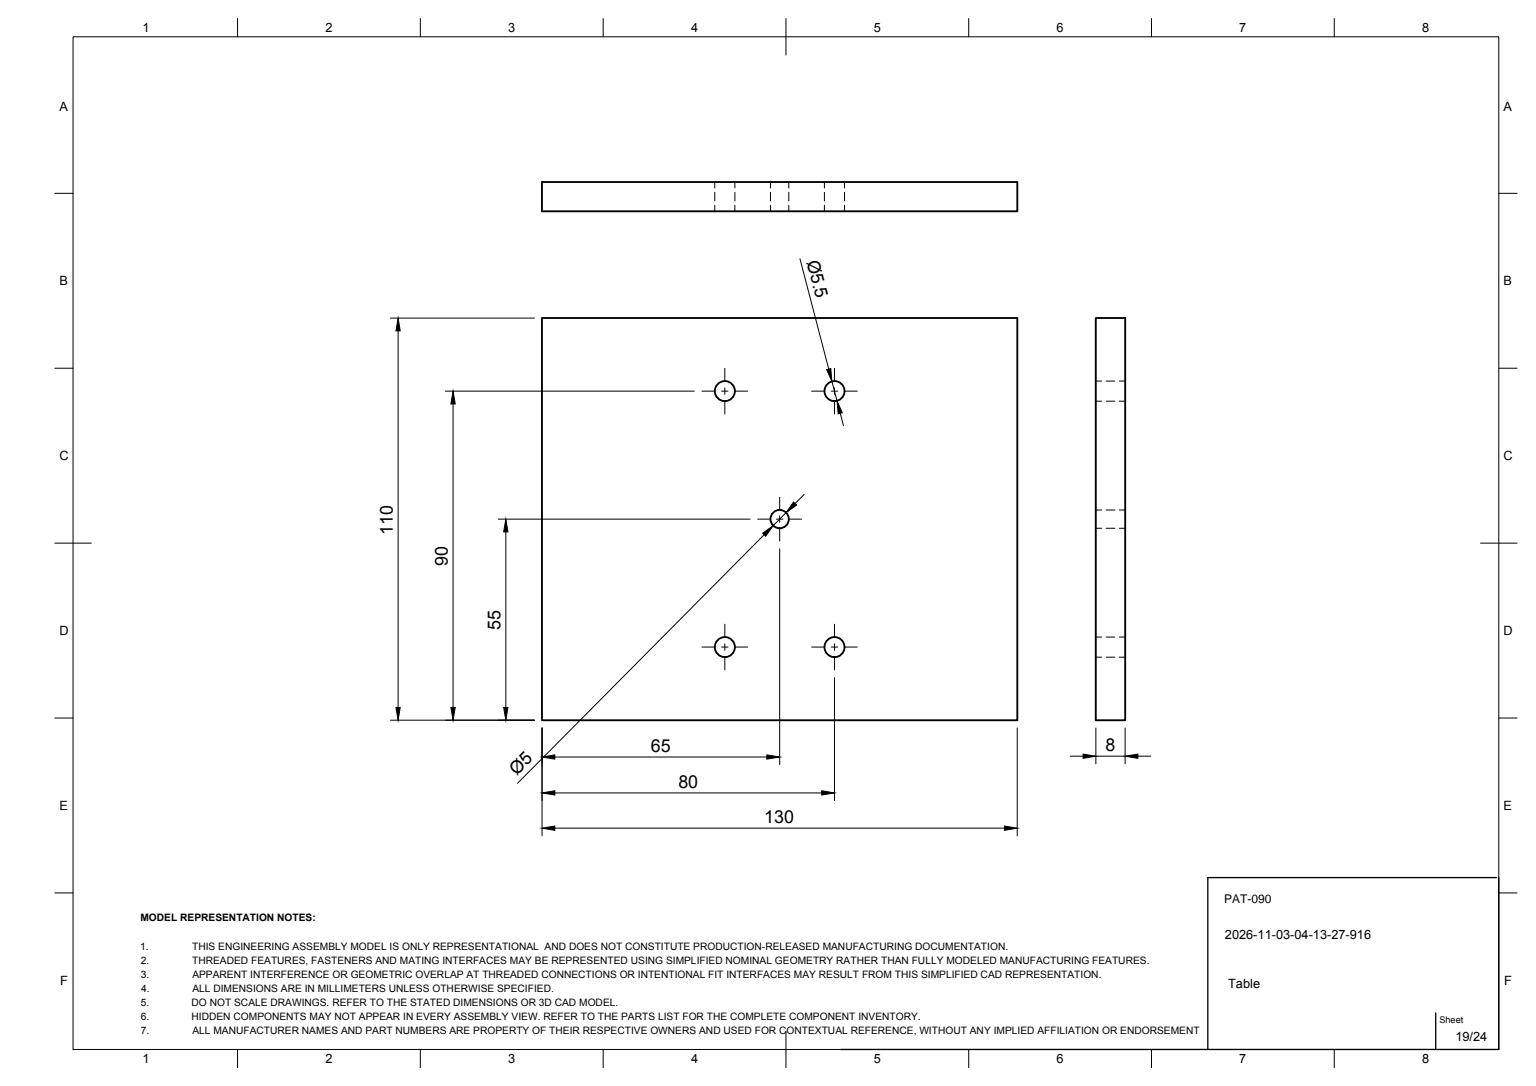
ISO-10303-21;
HEADER;
/* Generated by software containing ST-Developer
 * from STEP Tools, Inc. (www.steptools.com) 
 */

FILE_DESCRIPTION(
/* description */ ('Round-Shaft Linear Stage with Ball Bushings'),
/* implementation_level */ '2;1');

FILE_NAME(
/* name */ 'Table.step',
/* time_stamp */ '2026-10-27T10:47:55-07:00',
/* author */ (''),
/* organization */ (''),
/* preprocessor_version */ 'ST-DEVELOPER v20.2',
/* originating_system */ 'Autodesk Translation Framework v15.17.0.0',
/* authorisation */ '');

FILE_SCHEMA (('AUTOMOTIVE_DESIGN { 1 0 10303 214 3 1 1 }'));
ENDSEC;

DATA;
#10=MECHANICAL_DESIGN_GEOMETRIC_PRESENTATION_REPRESENTATION('',(#315),#7835);
#273=SHAPE_REPRESENTATION_RELATIONSHIP('SRR','None',#7962,#294);
#294=ADVANCED_BREP_SHAPE_REPRESENTATION('',(#335),#7826);
#315=STYLED_ITEM('',(#8158),#335);
#335=MANIFOLD_SOLID_BREP('Body1',#4406);
#431=FACE_BOUND('',#1136,.T.);
#432=FACE_BOUND('',#1137,.T.);
#433=FACE_BOUND('',#1138,.T.);
#434=FACE_BOUND('',#1139,.T.);
#435=FACE_BOUND('',#1140,.T.);
#436=FACE_BOUND('',#1142,.T.);
#437=FACE_BOUND('',#1143,.T.);
#438=FACE_BOUND('',#1144,.T.);
#439=FACE_BOUND('',#1145,.T.);
#440=FACE_BOUND('',#1146,.T.);
#556=PLANE('',#4968);
#557=PLANE('',#4969);
#558=PLANE('',#4970);
#559=PLANE('',#4971);
#560=PLANE('',#4972);
#561=PLANE('',#4973);
#778=FACE_OUTER_BOUND('',#1126,.T.);
#779=FACE_OUTER_BOUND('',#1127,.T.);
#780=FACE_OUTER_BOUND('',#1128,.T.);
#781=FACE_OUTER_BOUND('',#1129,.T.);
#782=FACE_OUTER_BOUND('',#1130,.T.);
#783=FACE_OUTER_BOUND('',#1131,.T.);
#784=FACE_OUTER_BOUND('',#1132,.T.);
#785=FACE_OUTER_BOUND('',#1133,.T.);
#786=FACE_OUTER_BOUND('',#1134,.T.);
#787=FACE_OUTER_BOUND('',#1135,.T.);
#788=FACE_OUTER_BOUND('',#1141,.T.);
#1126=EDGE_LOOP('',(#3686,#3687,#3688,#3689));
#1127=EDGE_LOOP('',(#3690,#3691,#3692,#3693));
#1128=EDGE_LOOP('',(#3694,#3695,#3696,#3697));
#1129=EDGE_LOOP('',(#3698,#3699,#3700,#3701));
#1130=EDGE_LOOP('',(#3702,#3703,#3704,#3705));
#1131=EDGE_LOOP('',(#3706,#3707,#3708,#3709));
#1132=EDGE_LOOP('',(#3710,#3711,#3712,#3713));
#1133=EDGE_LOOP('',(#3714,#3715,#3716,#3717));
#1134=EDGE_LOOP('',(#3718,#3719,#3720,#3721));
#1135=EDGE_LOOP('',(#3722,#3723,#3724,#3725));
#1136=EDGE_LOOP('',(#3726));
#1137=EDGE_LOOP('',(#3727));
#1138=EDGE_LOOP('',(#3728));
#1139=EDGE_LOOP('',(#3729));
#1140=EDGE_LOOP('',(#3730));
#1141=EDGE_LOOP('',(#3731,#3732,#3733,#3734));
#1142=EDGE_LOOP('',(#3735));
#1143=EDGE_LOOP('',(#3736));
#1144=EDGE_LOOP('',(#3737));
#1145=EDGE_LOOP('',(#3738));
#1146=EDGE_LOOP('',(#3739));
#1470=LINE('',#7328,#1810);
#1471=LINE('',#7334,#1811);
#1472=LINE('',#7340,#1812);
#1473=LINE('',#7346,#1813);
#1474=LINE('',#7352,#1814);
#1475=LINE('',#7357,#1815);
#1476=LINE('',#7359,#1816);
#1477=LINE('',#7361,#1817);
#1478=LINE('',#7362,#1818);
#1479=LINE('',#7365,#1819);
#1480=LINE('',#7367,#1820);
#1481=LINE('',#7368,#1821);
#1482=LINE('',#7371,#1822);
#1483=LINE('',#7373,#1823);
#1484=LINE('',#7374,#1824);
#1485=LINE('',#7376,#1825);
#1486=LINE('',#7377,#1826);
#1810=VECTOR('',#6009,0.25);
#1811=VECTOR('',#6016,0.274999999999999);
#1812=VECTOR('',#6023,0.275);
#1813=VECTOR('',#6030,0.275);
#1814=VECTOR('',#6037,0.274999999999999);
#1815=VECTOR('',#6042,1.);
#1816=VECTOR('',#6043,1.);
#1817=VECTOR('',#6044,1.);
#1818=VECTOR('',#6045,1.);
#1819=VECTOR('',#6048,1.);
#1820=VECTOR('',#6049,1.);
#1821=VECTOR('',#6050,1.);
#1822=VECTOR('',#6053,1.);
#1823=VECTOR('',#6054,1.);
#1824=VECTOR('',#6055,1.);
#1825=VECTOR('',#6058,1.);
#1826=VECTOR('',#6059,1.);
#2054=CIRCLE('',#4954,0.25);
#2055=CIRCLE('',#4955,0.25);
#2056=CIRCLE('',#4957,0.274999999999999);
#2057=CIRCLE('',#4958,0.274999999999999);
#2058=CIRCLE('',#4960,0.275);
#2059=CIRCLE('',#4961,0.275);
#2060=CIRCLE('',#4963,0.275);
#2061=CIRCLE('',#4964,0.275);
#2062=CIRCLE('',#4966,0.274999999999999);
#2063=CIRCLE('',#4967,0.274999999999999);
#2347=VERTEX_POINT('',#7325);
#2348=VERTEX_POINT('',#7327);
#2349=VERTEX_POINT('',#7331);
#2350=VERTEX_POINT('',#7333);
#2351=VERTEX_POINT('',#7337);
#2352=VERTEX_POINT('',#7339);
#2353=VERTEX_POINT('',#7343);
#2354=VERTEX_POINT('',#7345);
#2355=VERTEX_POINT('',#7349);
#2356=VERTEX_POINT('',#7351);
#2357=VERTEX_POINT('',#7355);
#2358=VERTEX_POINT('',#7356);
#2359=VERTEX_POINT('',#7358);
#2360=VERTEX_POINT('',#7360);
#2361=VERTEX_POINT('',#7364);
#2362=VERTEX_POINT('',#7366);
#2363=VERTEX_POINT('',#7370);
#2364=VERTEX_POINT('',#7372);
#2811=EDGE_CURVE('',#2347,#2347,#2054,.T.);
#2812=EDGE_CURVE('',#2347,#2348,#1470,.T.);
#2813=EDGE_CURVE('',#2348,#2348,#2055,.T.);
#2814=EDGE_CURVE('',#2349,#2349,#2056,.T.);
#2815=EDGE_CURVE('',#2349,#2350,#1471,.T.);
#2816=EDGE_CURVE('',#2350,#2350,#2057,.T.);
#2817=EDGE_CURVE('',#2351,#2351,#2058,.T.);
#2818=EDGE_CURVE('',#2351,#2352,#1472,.T.);
#2819=EDGE_CURVE('',#2352,#2352,#2059,.T.);
#2820=EDGE_CURVE('',#2353,#2353,#2060,.T.);
#2821=EDGE_CURVE('',#2353,#2354,#1473,.T.);
#2822=EDGE_CURVE('',#2354,#2354,#2061,.T.);
#2823=EDGE_CURVE('',#2355,#2355,#2062,.T.);
#2824=EDGE_CURVE('',#2355,#2356,#1474,.T.);
#2825=EDGE_CURVE('',#2356,#2356,#2063,.T.);
#2826=EDGE_CURVE('',#2357,#2358,#1475,.T.);
#2827=EDGE_CURVE('',#2358,#2359,#1476,.T.);
#2828=EDGE_CURVE('',#2360,#2359,#1477,.T.);
#2829=EDGE_CURVE('',#2357,#2360,#1478,.T.);
#2830=EDGE_CURVE('',#2361,#2357,#1479,.T.);
#2831=EDGE_CURVE('',#2362,#2360,#1480,.T.);
#2832=EDGE_CURVE('',#2361,#2362,#1481,.T.);
#2833=EDGE_CURVE('',#2363,#2361,#1482,.T.);
#2834=EDGE_CURVE('',#2364,#2362,#1483,.T.);
#2835=EDGE_CURVE('',#2363,#2364,#1484,.T.);
#2836=EDGE_CURVE('',#2358,#2363,#1485,.T.);
#2837=EDGE_CURVE('',#2359,#2364,#1486,.T.);
#3686=ORIENTED_EDGE('',*,*,#2811,.F.);
#3687=ORIENTED_EDGE('',*,*,#2812,.T.);
#3688=ORIENTED_EDGE('',*,*,#2813,.F.);
#3689=ORIENTED_EDGE('',*,*,#2812,.F.);
#3690=ORIENTED_EDGE('',*,*,#2814,.F.);
#3691=ORIENTED_EDGE('',*,*,#2815,.T.);
#3692=ORIENTED_EDGE('',*,*,#2816,.F.);
#3693=ORIENTED_EDGE('',*,*,#2815,.F.);
#3694=ORIENTED_EDGE('',*,*,#2817,.F.);
#3695=ORIENTED_EDGE('',*,*,#2818,.T.);
#3696=ORIENTED_EDGE('',*,*,#2819,.F.);
#3697=ORIENTED_EDGE('',*,*,#2818,.F.);
#3698=ORIENTED_EDGE('',*,*,#2820,.F.);
#3699=ORIENTED_EDGE('',*,*,#2821,.T.);
#3700=ORIENTED_EDGE('',*,*,#2822,.F.);
#3701=ORIENTED_EDGE('',*,*,#2821,.F.);
#3702=ORIENTED_EDGE('',*,*,#2823,.F.);
#3703=ORIENTED_EDGE('',*,*,#2824,.T.);
#3704=ORIENTED_EDGE('',*,*,#2825,.F.);
#3705=ORIENTED_EDGE('',*,*,#2824,.F.);
#3706=ORIENTED_EDGE('',*,*,#2826,.T.);
#3707=ORIENTED_EDGE('',*,*,#2827,.T.);
#3708=ORIENTED_EDGE('',*,*,#2828,.F.);
#3709=ORIENTED_EDGE('',*,*,#2829,.F.);
#3710=ORIENTED_EDGE('',*,*,#2830,.T.);
#3711=ORIENTED_EDGE('',*,*,#2829,.T.);
#3712=ORIENTED_EDGE('',*,*,#2831,.F.);
#3713=ORIENTED_EDGE('',*,*,#2832,.F.);
#3714=ORIENTED_EDGE('',*,*,#2833,.T.);
#3715=ORIENTED_EDGE('',*,*,#2832,.T.);
#3716=ORIENTED_EDGE('',*,*,#2834,.F.);
#3717=ORIENTED_EDGE('',*,*,#2835,.F.);
#3718=ORIENTED_EDGE('',*,*,#2836,.T.);
#3719=ORIENTED_EDGE('',*,*,#2835,.T.);
#3720=ORIENTED_EDGE('',*,*,#2837,.F.);
#3721=ORIENTED_EDGE('',*,*,#2827,.F.);
#3722=ORIENTED_EDGE('',*,*,#2837,.T.);
#3723=ORIENTED_EDGE('',*,*,#2834,.T.);
#3724=ORIENTED_EDGE('',*,*,#2831,.T.);
#3725=ORIENTED_EDGE('',*,*,#2828,.T.);
#3726=ORIENTED_EDGE('',*,*,#2813,.T.);
#3727=ORIENTED_EDGE('',*,*,#2816,.T.);
#3728=ORIENTED_EDGE('',*,*,#2819,.T.);
#3729=ORIENTED_EDGE('',*,*,#2822,.T.);
#3730=ORIENTED_EDGE('',*,*,#2825,.T.);
#3731=ORIENTED_EDGE('',*,*,#2836,.F.);
#3732=ORIENTED_EDGE('',*,*,#2826,.F.);
#3733=ORIENTED_EDGE('',*,*,#2830,.F.);
#3734=ORIENTED_EDGE('',*,*,#2833,.F.);
#3735=ORIENTED_EDGE('',*,*,#2811,.T.);
#3736=ORIENTED_EDGE('',*,*,#2814,.T.);
#3737=ORIENTED_EDGE('',*,*,#2817,.T.);
#3738=ORIENTED_EDGE('',*,*,#2820,.T.);
#3739=ORIENTED_EDGE('',*,*,#2823,.T.);
#4112=CYLINDRICAL_SURFACE('',#4953,0.25);
#4113=CYLINDRICAL_SURFACE('',#4956,0.274999999999999);
#4114=CYLINDRICAL_SURFACE('',#4959,0.275);
#4115=CYLINDRICAL_SURFACE('',#4962,0.275);
#4116=CYLINDRICAL_SURFACE('',#4965,0.274999999999999);
#4297=ADVANCED_FACE('',(#778),#4112,.F.);
#4298=ADVANCED_FACE('',(#779),#4113,.F.);
#4299=ADVANCED_FACE('',(#780),#4114,.F.);
#4300=ADVANCED_FACE('',(#781),#4115,.F.);
#4301=ADVANCED_FACE('',(#782),#4116,.F.);
#4302=ADVANCED_FACE('',(#783),#556,.T.);
#4303=ADVANCED_FACE('',(#784),#557,.T.);
#4304=ADVANCED_FACE('',(#785),#558,.T.);
#4305=ADVANCED_FACE('',(#786),#559,.T.);
#4306=ADVANCED_FACE('',(#787,#431,#432,#433,#434,#435),#560,.T.);
#4307=ADVANCED_FACE('',(#788,#436,#437,#438,#439,#440),#561,.F.);
#4406=CLOSED_SHELL('',(#4297,#4298,#4299,#4300,#4301,#4302,#4303,#4304,
#4305,#4306,#4307));
#4952=AXIS2_PLACEMENT_3D('',#7323,#6003,#6004);
#4953=AXIS2_PLACEMENT_3D('',#7324,#6005,#6006);
#4954=AXIS2_PLACEMENT_3D('',#7326,#6007,#6008);
#4955=AXIS2_PLACEMENT_3D('',#7329,#6010,#6011);
#4956=AXIS2_PLACEMENT_3D('',#7330,#6012,#6013);
#4957=AXIS2_PLACEMENT_3D('',#7332,#6014,#6015);
#4958=AXIS2_PLACEMENT_3D('',#7335,#6017,#6018);
#4959=AXIS2_PLACEMENT_3D('',#7336,#6019,#6020);
#4960=AXIS2_PLACEMENT_3D('',#7338,#6021,#6022);
#4961=AXIS2_PLACEMENT_3D('',#7341,#6024,#6025);
#4962=AXIS2_PLACEMENT_3D('',#7342,#6026,#6027);
#4963=AXIS2_PLACEMENT_3D('',#7344,#6028,#6029);
#4964=AXIS2_PLACEMENT_3D('',#7347,#6031,#6032);
#4965=AXIS2_PLACEMENT_3D('',#7348,#6033,#6034);
#4966=AXIS2_PLACEMENT_3D('',#7350,#6035,#6036);
#4967=AXIS2_PLACEMENT_3D('',#7353,#6038,#6039);
#4968=AXIS2_PLACEMENT_3D('',#7354,#6040,#6041);
#4969=AXIS2_PLACEMENT_3D('',#7363,#6046,#6047);
#4970=AXIS2_PLACEMENT_3D('',#7369,#6051,#6052);
#4971=AXIS2_PLACEMENT_3D('',#7375,#6056,#6057);
#4972=AXIS2_PLACEMENT_3D('',#7378,#6060,#6061);
#4973=AXIS2_PLACEMENT_3D('',#7379,#6062,#6063);
#6003=DIRECTION('axis',(0.,0.,1.));
#6004=DIRECTION('refdir',(1.,0.,0.));
#6005=DIRECTION('center_axis',(0.,0.,1.));
#6006=DIRECTION('ref_axis',(1.,0.,0.));
#6007=DIRECTION('center_axis',(0.,0.,1.));
#6008=DIRECTION('ref_axis',(1.,0.,0.));
#6009=DIRECTION('',(0.,0.,1.));
#6010=DIRECTION('center_axis',(0.,0.,-1.));
#6011=DIRECTION('ref_axis',(1.,0.,0.));
#6012=DIRECTION('center_axis',(0.,0.,1.));
#6013=DIRECTION('ref_axis',(1.,0.,0.));
#6014=DIRECTION('center_axis',(0.,0.,1.));
#6015=DIRECTION('ref_axis',(1.,0.,0.));
#6016=DIRECTION('',(0.,0.,1.));
#6017=DIRECTION('center_axis',(0.,0.,-1.));
#6018=DIRECTION('ref_axis',(1.,0.,0.));
#6019=DIRECTION('center_axis',(0.,0.,1.));
#6020=DIRECTION('ref_axis',(1.,0.,0.));
#6021=DIRECTION('center_axis',(0.,0.,1.));
#6022=DIRECTION('ref_axis',(1.,0.,0.));
#6023=DIRECTION('',(0.,0.,1.));
#6024=DIRECTION('center_axis',(0.,0.,-1.));
#6025=DIRECTION('ref_axis',(1.,0.,0.));
#6026=DIRECTION('center_axis',(0.,0.,1.));
#6027=DIRECTION('ref_axis',(1.,0.,0.));
#6028=DIRECTION('center_axis',(0.,0.,1.));
#6029=DIRECTION('ref_axis',(1.,0.,0.));
#6030=DIRECTION('',(0.,0.,1.));
#6031=DIRECTION('center_axis',(0.,0.,-1.));
#6032=DIRECTION('ref_axis',(1.,0.,0.));
#6033=DIRECTION('center_axis',(0.,0.,1.));
#6034=DIRECTION('ref_axis',(1.,0.,0.));
#6035=DIRECTION('center_axis',(0.,0.,1.));
#6036=DIRECTION('ref_axis',(1.,0.,0.));
#6037=DIRECTION('',(0.,0.,1.));
#6038=DIRECTION('center_axis',(0.,0.,-1.));
#6039=DIRECTION('ref_axis',(1.,0.,0.));
#6040=DIRECTION('center_axis',(0.,1.,0.));
#6041=DIRECTION('ref_axis',(-1.,0.,0.));
#6042=DIRECTION('',(-1.,0.,0.));
#6043=DIRECTION('',(0.,0.,1.));
#6044=DIRECTION('',(-1.,0.,0.));
#6045=DIRECTION('',(0.,0.,1.));
#6046=DIRECTION('center_axis',(1.,0.,0.));
#6047=DIRECTION('ref_axis',(0.,1.,0.));
#6048=DIRECTION('',(0.,1.,0.));
#6049=DIRECTION('',(0.,1.,0.));
#6050=DIRECTION('',(0.,0.,1.));
#6051=DIRECTION('center_axis',(0.,-1.,0.));
#6052=DIRECTION('ref_axis',(1.,0.,0.));
#6053=DIRECTION('',(1.,0.,0.));
#6054=DIRECTION('',(1.,0.,0.));
#6055=DIRECTION('',(0.,0.,1.));
#6056=DIRECTION('center_axis',(-1.,0.,0.));
#6057=DIRECTION('ref_axis',(0.,-1.,0.));
#6058=DIRECTION('',(0.,-1.,0.));
#6059=DIRECTION('',(0.,-1.,0.));
#6060=DIRECTION('center_axis',(0.,0.,1.));
#6061=DIRECTION('ref_axis',(1.,0.,0.));
#6062=DIRECTION('center_axis',(0.,0.,1.));
#6063=DIRECTION('ref_axis',(1.,0.,0.));
#7323=CARTESIAN_POINT('',(0.,0.,0.));
#7324=CARTESIAN_POINT('Origin',(15.,0.,5.7));
#7325=CARTESIAN_POINT('',(14.75,-3.06161699786838E-17,5.8));
#7326=CARTESIAN_POINT('Origin',(15.,0.,5.8));
#7327=CARTESIAN_POINT('',(14.75,3.06161699786838E-17,6.6));
#7328=CARTESIAN_POINT('',(14.75,-3.06161699786838E-17,5.7));
#7329=CARTESIAN_POINT('Origin',(15.,0.,6.6));
#7330=CARTESIAN_POINT('Origin',(18.5,-1.5,5.7));
#7331=CARTESIAN_POINT('',(18.225,-1.5,5.8));
#7332=CARTESIAN_POINT('Origin',(18.5,-1.5,5.8));
#7333=CARTESIAN_POINT('',(18.225,-1.5,6.6));
#7334=CARTESIAN_POINT('',(18.225,-1.5,5.7));
#7335=CARTESIAN_POINT('Origin',(18.5,-1.5,6.6));
#7336=CARTESIAN_POINT('Origin',(11.5,1.5,5.7));
#7337=CARTESIAN_POINT('',(11.225,1.5,5.8));
#7338=CARTESIAN_POINT('Origin',(11.5,1.5,5.8));
#7339=CARTESIAN_POINT('',(11.225,1.5,6.6));
#7340=CARTESIAN_POINT('',(11.225,1.5,5.7));
#7341=CARTESIAN_POINT('Origin',(11.5,1.5,6.6));
#7342=CARTESIAN_POINT('Origin',(11.5,-1.5,5.7));
#7343=CARTESIAN_POINT('',(11.225,-1.5,5.8));
#7344=CARTESIAN_POINT('Origin',(11.5,-1.5,5.8));
#7345=CARTESIAN_POINT('',(11.225,-1.5,6.6));
#7346=CARTESIAN_POINT('',(11.225,-1.5,5.7));
#7347=CARTESIAN_POINT('Origin',(11.5,-1.5,6.6));
#7348=CARTESIAN_POINT('Origin',(18.5,1.5,5.7));
#7349=CARTESIAN_POINT('',(18.225,1.5,5.8));
#7350=CARTESIAN_POINT('Origin',(18.5,1.5,5.8));
#7351=CARTESIAN_POINT('',(18.225,1.5,6.6));
#7352=CARTESIAN_POINT('',(18.225,1.5,5.7));
#7353=CARTESIAN_POINT('Origin',(18.5,1.5,6.6));
#7354=CARTESIAN_POINT('Origin',(20.5,6.5,5.8));
#7355=CARTESIAN_POINT('',(20.5,6.5,5.8));
#7356=CARTESIAN_POINT('',(9.5,6.5,5.8));
#7357=CARTESIAN_POINT('',(20.5,6.5,5.8));
#7358=CARTESIAN_POINT('',(9.5,6.5,6.6));
#7359=CARTESIAN_POINT('',(9.5,6.5,5.8));
#7360=CARTESIAN_POINT('',(20.5,6.5,6.6));
#7361=CARTESIAN_POINT('',(20.5,6.5,6.6));
#7362=CARTESIAN_POINT('',(20.5,6.5,5.8));
#7363=CARTESIAN_POINT('Origin',(20.5,-6.5,5.8));
#7364=CARTESIAN_POINT('',(20.5,-6.5,5.8));
#7365=CARTESIAN_POINT('',(20.5,-6.5,5.8));
#7366=CARTESIAN_POINT('',(20.5,-6.5,6.6));
#7367=CARTESIAN_POINT('',(20.5,-6.5,6.6));
#7368=CARTESIAN_POINT('',(20.5,-6.5,5.8));
#7369=CARTESIAN_POINT('Origin',(9.5,-6.5,5.8));
#7370=CARTESIAN_POINT('',(9.5,-6.5,5.8));
#7371=CARTESIAN_POINT('',(9.5,-6.5,5.8));
#7372=CARTESIAN_POINT('',(9.5,-6.5,6.6));
#7373=CARTESIAN_POINT('',(9.5,-6.5,6.6));
#7374=CARTESIAN_POINT('',(9.5,-6.5,5.8));
#7375=CARTESIAN_POINT('Origin',(9.5,6.5,5.8));
#7376=CARTESIAN_POINT('',(9.5,6.5,5.8));
#7377=CARTESIAN_POINT('',(9.5,6.5,6.6));
#7378=CARTESIAN_POINT('Origin',(15.,0.,6.6));
#7379=CARTESIAN_POINT('Origin',(15.,0.,5.8));
#7800=UNCERTAINTY_MEASURE_WITH_UNIT(LENGTH_MEASURE(0.001),#7836,
'DISTANCE_ACCURACY_VALUE',
'Maximum model space distance between geometric entities at asserted c
onnectivities');
#7809=UNCERTAINTY_MEASURE_WITH_UNIT(LENGTH_MEASURE(0.001),#7836,
'DISTANCE_ACCURACY_VALUE',
'Maximum model space distance between geometric entities at asserted c
onnectivities');
#7826=(
GEOMETRIC_REPRESENTATION_CONTEXT(3)
GLOBAL_UNCERTAINTY_ASSIGNED_CONTEXT((#7800))
GLOBAL_UNIT_ASSIGNED_CONTEXT((#7836,#7838,#7839))
REPRESENTATION_CONTEXT('','3D')
);
#7835=(
GEOMETRIC_REPRESENTATION_CONTEXT(3)
GLOBAL_UNCERTAINTY_ASSIGNED_CONTEXT((#7809))
GLOBAL_UNIT_ASSIGNED_CONTEXT((#7836,#7838,#7839))
REPRESENTATION_CONTEXT('','3D')
);
#7836=(
LENGTH_UNIT()
NAMED_UNIT(*)
SI_UNIT(.CENTI.,.METRE.)
);
#7838=(
NAMED_UNIT(*)
PLANE_ANGLE_UNIT()
SI_UNIT($,.RADIAN.)
);
#7839=(
NAMED_UNIT(*)
SI_UNIT($,.STERADIAN.)
SOLID_ANGLE_UNIT()
);
#7856=SHAPE_DEFINITION_REPRESENTATION(#7881,#7962);
#7881=PRODUCT_DEFINITION_SHAPE('',$,#7988);
#7962=SHAPE_REPRESENTATION('',(#4952),#7826);
#7971=PRODUCT_DEFINITION_CONTEXT('part definition',#8048,'design');
#7988=PRODUCT_DEFINITION('Table','Table',#8013,#7971);
#8013=PRODUCT_DEFINITION_FORMATION('',$,#8066);
#8048=APPLICATION_CONTEXT(
'Core Data for Automotive Mechanical Design Process');
#8049=PRODUCT_CONTEXT('part definition',#8048,'mechanical');
#8066=PRODUCT('Table','Table','Table',(#8049));
#8152=COLOUR_RGB('Off White',0.89,0.88,0.83);
#8153=FILL_AREA_STYLE_COLOUR('',#8152);
#8154=FILL_AREA_STYLE('',(#8153));
#8155=SURFACE_STYLE_FILL_AREA(#8154);
#8156=SURFACE_SIDE_STYLE('',(#8155));
#8157=SURFACE_STYLE_USAGE(.BOTH.,#8156);
#8158=PRESENTATION_STYLE_ASSIGNMENT((#8157));
ENDSEC;
END-ISO-10303-21;
